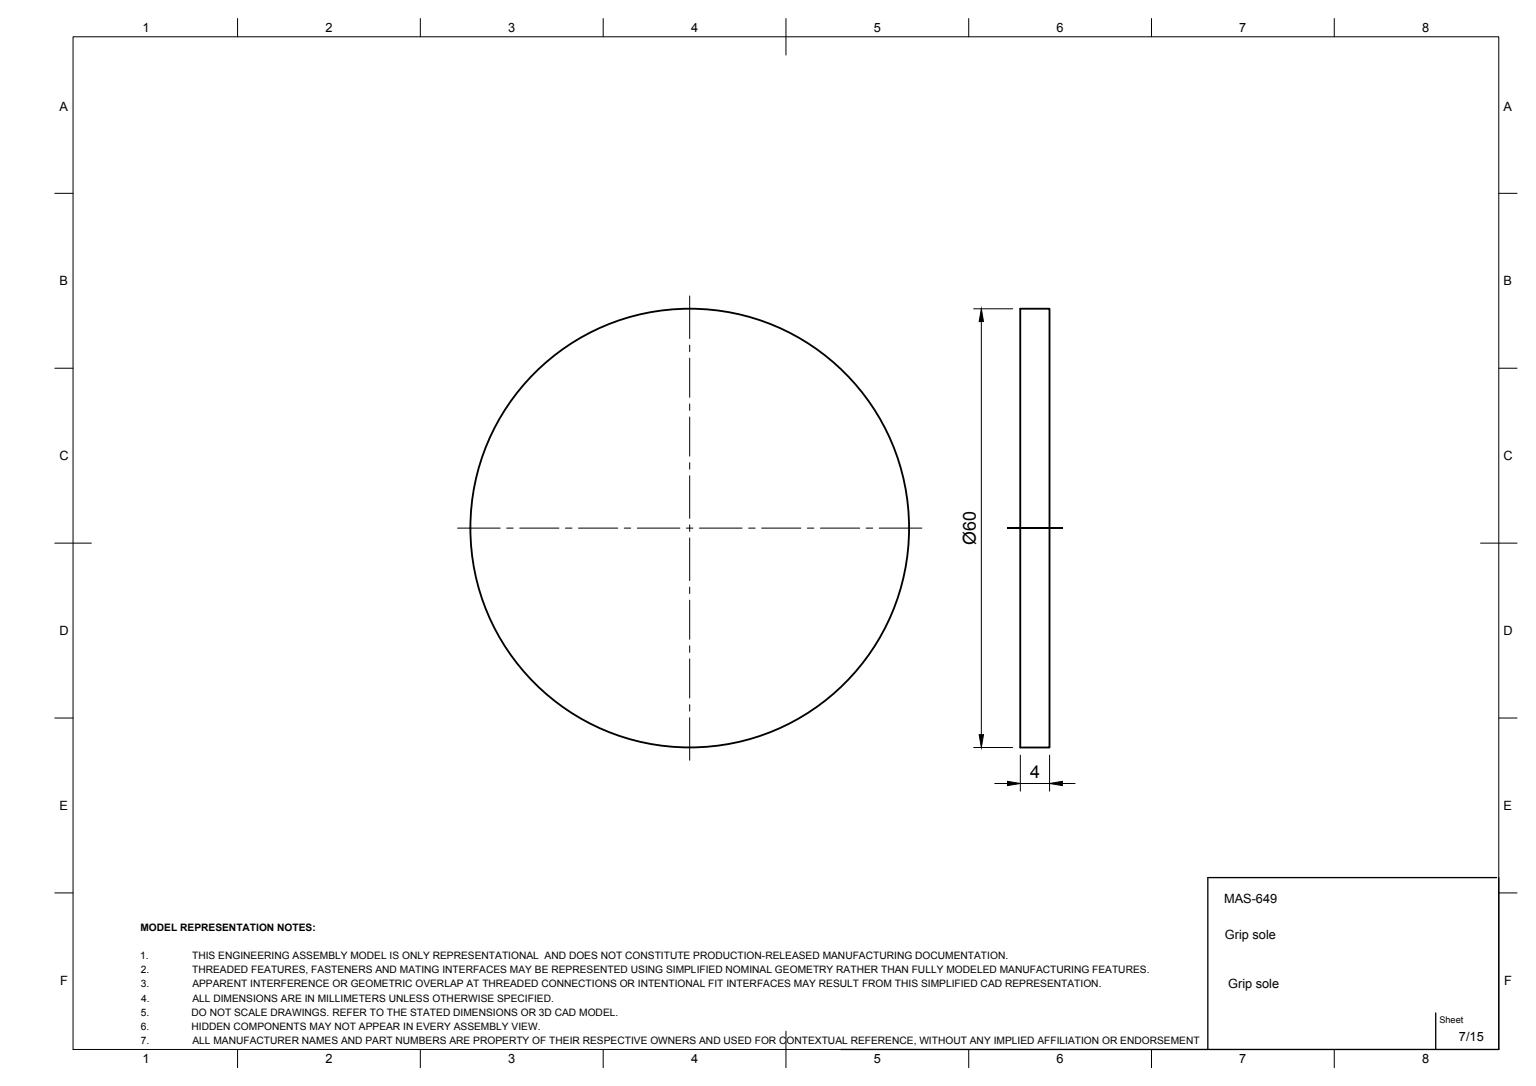
ISO-10303-21;
HEADER;
/* Generated by software containing ST-Developer
 * from STEP Tools, Inc. (www.steptools.com) 
 */

FILE_DESCRIPTION(
/* description */ ('Independent equipment support assembly with bolted 600 x 500 mm welde
d perimeter frame, four adjustable legs and swivel feet. Nominal overa
ll height 518 mm. No load rating assigned.'),
/* implementation_level */ '2;1');

FILE_NAME(
/* name */ 'Grip sole.step',
/* time_stamp */ '2026-11-07T17:30:39-08:00',
/* author */ (''),
/* organization */ (''),
/* preprocessor_version */ 'ST-DEVELOPER v20.2',
/* originating_system */ 'Autodesk Translation Framework v15.17.0.0',
/* authorisation */ '');

FILE_SCHEMA (('AUTOMOTIVE_DESIGN { 1 0 10303 214 3 1 1 }'));
ENDSEC;

DATA;
#10=MECHANICAL_DESIGN_GEOMETRIC_PRESENTATION_REPRESENTATION('',(#2216),#63755);
#425=CIRCLE('',#15141,30.);
#426=CIRCLE('',#15142,30.);
#1937=CYLINDRICAL_SURFACE('',#15140,30.);
#2184=SHAPE_REPRESENTATION_RELATIONSHIP('SRR','None',#63869,#2200);
#2200=ADVANCED_BREP_SHAPE_REPRESENTATION('',(#2232),#63747);
#2216=STYLED_ITEM('',(#63960),#2232);
#2232=MANIFOLD_SOLID_BREP('Body1',#14317);
#2765=FACE_OUTER_BOUND('',#3566,.T.);
#2766=FACE_OUTER_BOUND('',#3567,.T.);
#2767=FACE_OUTER_BOUND('',#3568,.T.);
#3566=EDGE_LOOP('',(#11761,#11762,#11763,#11764));
#3567=EDGE_LOOP('',(#11765));
#3568=EDGE_LOOP('',(#11766));
#4437=LINE('',#47149,#5273);
#5273=VECTOR('',#17346,30.);
#6436=VERTEX_POINT('',#47146);
#6437=VERTEX_POINT('',#47148);
#8303=EDGE_CURVE('',#6436,#6436,#425,.T.);
#8304=EDGE_CURVE('',#6436,#6437,#4437,.T.);
#8305=EDGE_CURVE('',#6437,#6437,#426,.T.);
#11761=ORIENTED_EDGE('',*,*,#8303,.F.);
#11762=ORIENTED_EDGE('',*,*,#8304,.T.);
#11763=ORIENTED_EDGE('',*,*,#8305,.T.);
#11764=ORIENTED_EDGE('',*,*,#8304,.F.);
#11765=ORIENTED_EDGE('',*,*,#8303,.T.);
#11766=ORIENTED_EDGE('',*,*,#8305,.F.);
#13506=PLANE('',#15143);
#13507=PLANE('',#15144);
#14011=ADVANCED_FACE('',(#2765),#1937,.T.);
#14012=ADVANCED_FACE('',(#2766),#13506,.T.);
#14013=ADVANCED_FACE('',(#2767),#13507,.F.);
#14317=CLOSED_SHELL('',(#14011,#14012,#14013));
#15139=AXIS2_PLACEMENT_3D('',#47144,#17340,#17341);
#15140=AXIS2_PLACEMENT_3D('',#47145,#17342,#17343);
#15141=AXIS2_PLACEMENT_3D('',#47147,#17344,#17345);
#15142=AXIS2_PLACEMENT_3D('',#47150,#17347,#17348);
#15143=AXIS2_PLACEMENT_3D('',#47151,#17349,#17350);
#15144=AXIS2_PLACEMENT_3D('',#47152,#17351,#17352);
#17340=DIRECTION('axis',(0.,0.,1.));
#17341=DIRECTION('refdir',(1.,0.,0.));
#17342=DIRECTION('center_axis',(0.,0.,1.));
#17343=DIRECTION('ref_axis',(1.,0.,0.));
#17344=DIRECTION('center_axis',(0.,0.,1.));
#17345=DIRECTION('ref_axis',(1.,0.,0.));
#17346=DIRECTION('',(0.,0.,-1.));
#17347=DIRECTION('center_axis',(0.,0.,1.));
#17348=DIRECTION('ref_axis',(1.,0.,0.));
#17349=DIRECTION('center_axis',(0.,0.,1.));
#17350=DIRECTION('ref_axis',(1.,0.,0.));
#17351=DIRECTION('center_axis',(0.,0.,1.));
#17352=DIRECTION('ref_axis',(1.,0.,0.));
#47144=CARTESIAN_POINT('',(0.,0.,0.));
#47145=CARTESIAN_POINT('Origin',(0.,0.,0.));
#47146=CARTESIAN_POINT('',(-30.,-3.67394039744206E-15,4.));
#47147=CARTESIAN_POINT('Origin',(0.,0.,4.));
#47148=CARTESIAN_POINT('',(-30.,-3.67394039744206E-15,0.));
#47149=CARTESIAN_POINT('',(-30.,-3.67394039744206E-15,0.));
#47150=CARTESIAN_POINT('Origin',(0.,0.,0.));
#47151=CARTESIAN_POINT('Origin',(0.,0.,4.));
#47152=CARTESIAN_POINT('Origin',(0.,0.,0.));
#63727=UNCERTAINTY_MEASURE_WITH_UNIT(LENGTH_MEASURE(0.01),#63756,
'DISTANCE_ACCURACY_VALUE',
'Maximum model space distance between geometric entities at asserted c
onnectivities');
#63735=UNCERTAINTY_MEASURE_WITH_UNIT(LENGTH_MEASURE(0.01),#63756,
'DISTANCE_ACCURACY_VALUE',
'Maximum model space distance between geometric entities at asserted c
onnectivities');
#63747=(
GEOMETRIC_REPRESENTATION_CONTEXT(3)
GLOBAL_UNCERTAINTY_ASSIGNED_CONTEXT((#63727))
GLOBAL_UNIT_ASSIGNED_CONTEXT((#63756,#63758,#63759))
REPRESENTATION_CONTEXT('','3D')
);
#63755=(
GEOMETRIC_REPRESENTATION_CONTEXT(3)
GLOBAL_UNCERTAINTY_ASSIGNED_CONTEXT((#63735))
GLOBAL_UNIT_ASSIGNED_CONTEXT((#63756,#63758,#63759))
REPRESENTATION_CONTEXT('','3D')
);
#63756=(
LENGTH_UNIT()
NAMED_UNIT(*)
SI_UNIT(.MILLI.,.METRE.)
);
#63758=(
NAMED_UNIT(*)
PLANE_ANGLE_UNIT()
SI_UNIT($,.RADIAN.)
);
#63759=(
NAMED_UNIT(*)
SI_UNIT($,.STERADIAN.)
SOLID_ANGLE_UNIT()
);
#63771=SHAPE_DEFINITION_REPRESENTATION(#63830,#63869);
#63830=PRODUCT_DEFINITION_SHAPE('',$,#63889);
#63869=SHAPE_REPRESENTATION('',(#15139),#63747);
#63877=PRODUCT_DEFINITION_CONTEXT('part definition',#63936,'design');
#63889=PRODUCT_DEFINITION('Grip sole','Grip sole',#63908,#63877);
#63908=PRODUCT_DEFINITION_FORMATION('',$,#63949);
#63936=APPLICATION_CONTEXT(
'Core Data for Automotive Mechanical Design Process');
#63937=PRODUCT_CONTEXT('part definition',#63936,'mechanical');
#63949=PRODUCT('Grip sole','Grip sole',
'Bonded elastomer sole; nominal diameter 60 mm, thickness 4 mm.',(#63937));
#63960=PRESENTATION_STYLE_ASSIGNMENT((#63967));
#63967=SURFACE_STYLE_USAGE(.BOTH.,#63974);
#63974=SURFACE_SIDE_STYLE('',(#63981));
#63981=SURFACE_STYLE_FILL_AREA(#63988);
#63988=FILL_AREA_STYLE('Dark gray',(#63995));
#63995=FILL_AREA_STYLE_COLOUR('Dark gray',#64002);
#64002=COLOUR_RGB('Dark gray',0.250980392156863,0.282352941176471,0.32156862745098);
ENDSEC;
END-ISO-10303-21;
